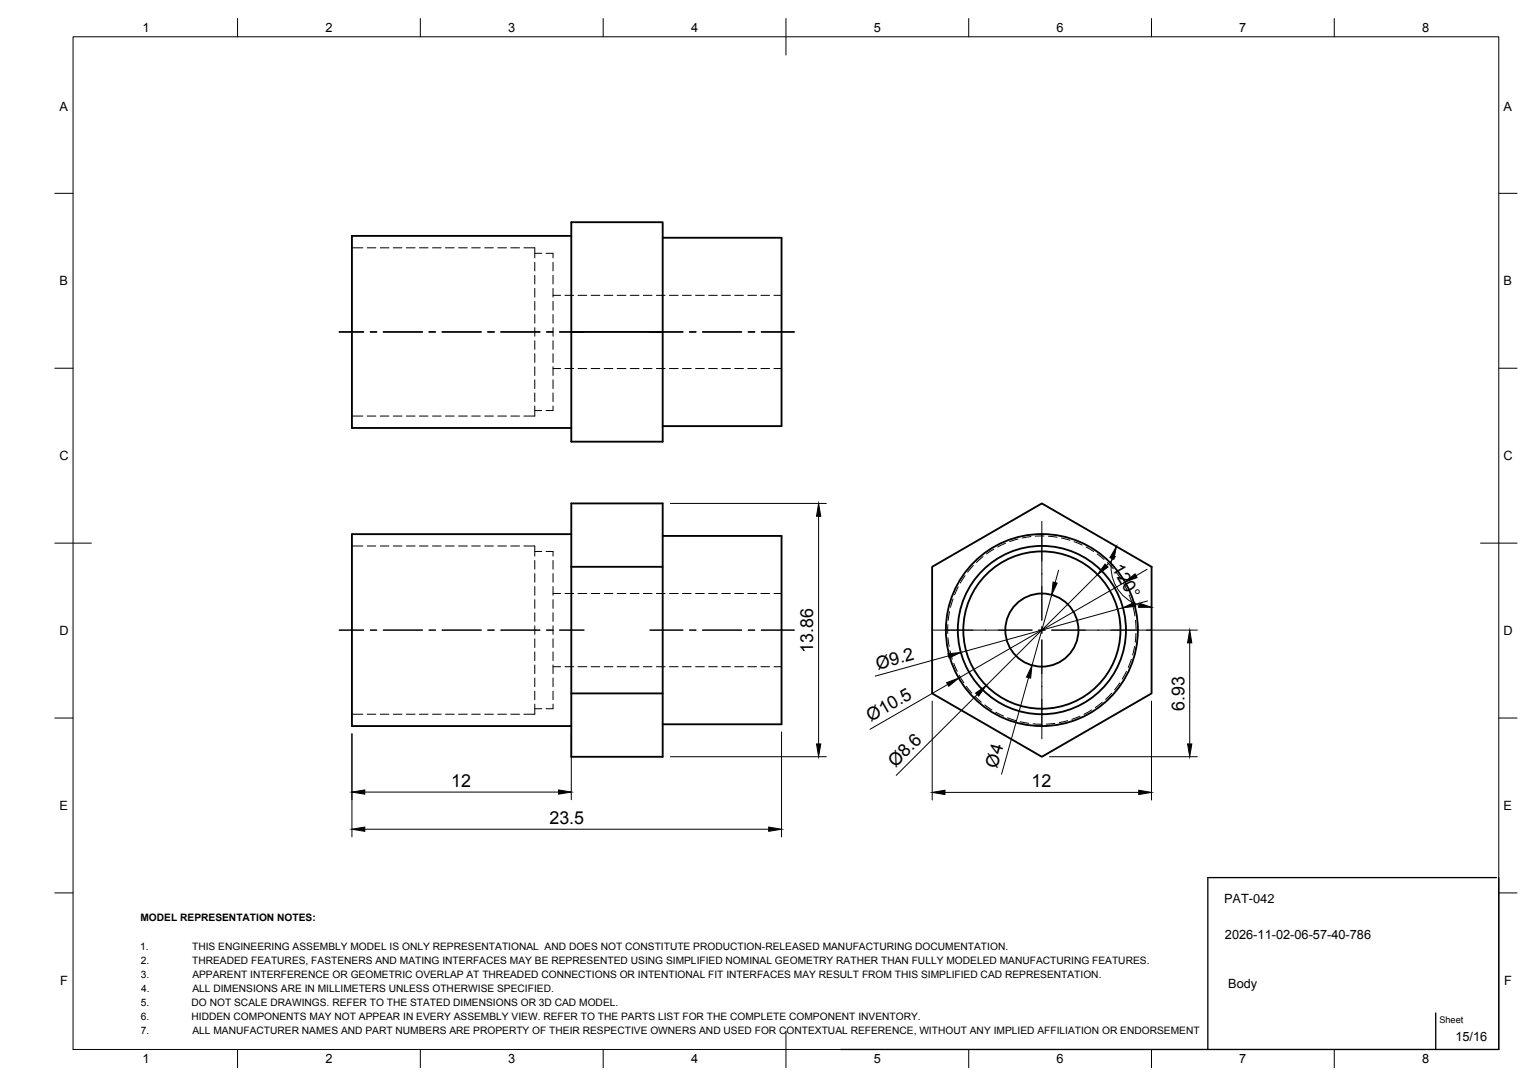
ISO-10303-21;
HEADER;
/* Generated by software containing ST-Developer
 * from STEP Tools, Inc. (www.steptools.com) 
 */

FILE_DESCRIPTION(
/* description */ ('Manifold and mounting hardware'),
/* implementation_level */ '2;1');

FILE_NAME(
/* name */ 'Body.step',
/* time_stamp */ '2026-10-28T21:46:49-07:00',
/* author */ (''),
/* organization */ (''),
/* preprocessor_version */ 'ST-DEVELOPER v20.2',
/* originating_system */ 'Autodesk Translation Framework v15.17.0.0',
/* authorisation */ '');

FILE_SCHEMA (('AUTOMOTIVE_DESIGN { 1 0 10303 214 3 1 1 }'));
ENDSEC;

DATA;
#10=MECHANICAL_DESIGN_GEOMETRIC_PRESENTATION_REPRESENTATION('',(#159),#5638);
#131=SHAPE_REPRESENTATION_RELATIONSHIP('SRR','None',#5711,#145);
#145=ADVANCED_BREP_SHAPE_REPRESENTATION('',(#173),#5633);
#159=STYLED_ITEM('',(#5839),#173);
#173=MANIFOLD_SOLID_BREP('Body1',#3149);
#241=FACE_BOUND('',#724,.T.);
#242=FACE_BOUND('',#726,.T.);
#243=FACE_BOUND('',#728,.T.);
#244=FACE_BOUND('',#736,.T.);
#245=FACE_BOUND('',#739,.T.);
#246=FACE_BOUND('',#743,.T.);
#318=CYLINDRICAL_SURFACE('',#3573,0.43);
#319=CYLINDRICAL_SURFACE('',#3590,0.46);
#320=CYLINDRICAL_SURFACE('',#3594,0.525);
#321=CYLINDRICAL_SURFACE('',#3595,0.515);
#322=CYLINDRICAL_SURFACE('',#3599,0.2);
#473=FACE_OUTER_BOUND('',#722,.T.);
#474=FACE_OUTER_BOUND('',#723,.T.);
#475=FACE_OUTER_BOUND('',#725,.T.);
#476=FACE_OUTER_BOUND('',#727,.T.);
#477=FACE_OUTER_BOUND('',#729,.T.);
#478=FACE_OUTER_BOUND('',#730,.T.);
#479=FACE_OUTER_BOUND('',#731,.T.);
#480=FACE_OUTER_BOUND('',#732,.T.);
#481=FACE_OUTER_BOUND('',#733,.T.);
#482=FACE_OUTER_BOUND('',#734,.T.);
#483=FACE_OUTER_BOUND('',#735,.T.);
#484=FACE_OUTER_BOUND('',#737,.T.);
#485=FACE_OUTER_BOUND('',#738,.T.);
#486=FACE_OUTER_BOUND('',#740,.T.);
#487=FACE_OUTER_BOUND('',#741,.T.);
#488=FACE_OUTER_BOUND('',#742,.T.);
#489=FACE_OUTER_BOUND('',#744,.T.);
#722=EDGE_LOOP('',(#2674,#2675,#2676,#2677));
#723=EDGE_LOOP('',(#2678));
#724=EDGE_LOOP('',(#2679));
#725=EDGE_LOOP('',(#2680,#2681,#2682,#2683,#2684,#2685));
#726=EDGE_LOOP('',(#2686));
#727=EDGE_LOOP('',(#2687,#2688,#2689,#2690,#2691,#2692));
#728=EDGE_LOOP('',(#2693));
#729=EDGE_LOOP('',(#2694,#2695,#2696,#2697));
#730=EDGE_LOOP('',(#2698,#2699,#2700,#2701));
#731=EDGE_LOOP('',(#2702,#2703,#2704,#2705));
#732=EDGE_LOOP('',(#2706,#2707,#2708,#2709));
#733=EDGE_LOOP('',(#2710,#2711,#2712,#2713));
#734=EDGE_LOOP('',(#2714,#2715,#2716,#2717));
#735=EDGE_LOOP('',(#2718));
#736=EDGE_LOOP('',(#2719));
#737=EDGE_LOOP('',(#2720,#2721,#2722,#2723));
#738=EDGE_LOOP('',(#2724));
#739=EDGE_LOOP('',(#2725));
#740=EDGE_LOOP('',(#2726,#2727,#2728,#2729));
#741=EDGE_LOOP('',(#2730,#2731,#2732,#2733));
#742=EDGE_LOOP('',(#2734));
#743=EDGE_LOOP('',(#2735));
#744=EDGE_LOOP('',(#2736,#2737,#2738,#2739));
#870=CIRCLE('',#3574,0.43);
#871=CIRCLE('',#3575,0.43);
#872=CIRCLE('',#3577,0.2);
#873=CIRCLE('',#3579,0.525);
#874=CIRCLE('',#3581,0.515);
#875=CIRCLE('',#3589,0.46);
#876=CIRCLE('',#3591,0.46);
#877=CIRCLE('',#3593,0.525);
#878=CIRCLE('',#3596,0.515);
#879=CIRCLE('',#3598,0.2);
#1099=LINE('',#5396,#1346);
#1100=LINE('',#5404,#1347);
#1101=LINE('',#5406,#1348);
#1102=LINE('',#5408,#1349);
#1103=LINE('',#5410,#1350);
#1104=LINE('',#5412,#1351);
#1105=LINE('',#5413,#1352);
#1106=LINE('',#5419,#1353);
#1107=LINE('',#5421,#1354);
#1108=LINE('',#5423,#1355);
#1109=LINE('',#5425,#1356);
#1110=LINE('',#5427,#1357);
#1111=LINE('',#5428,#1358);
#1112=LINE('',#5432,#1359);
#1113=LINE('',#5433,#1360);
#1114=LINE('',#5435,#1361);
#1115=LINE('',#5437,#1362);
#1116=LINE('',#5439,#1363);
#1117=LINE('',#5441,#1364);
#1118=LINE('',#5448,#1365);
#1119=LINE('',#5454,#1366);
#1120=LINE('',#5458,#1367);
#1121=LINE('',#5463,#1368);
#1346=VECTOR('',#4406,0.43);
#1347=VECTOR('',#4415,1.);
#1348=VECTOR('',#4416,1.);
#1349=VECTOR('',#4417,1.);
#1350=VECTOR('',#4418,1.);
#1351=VECTOR('',#4419,1.);
#1352=VECTOR('',#4420,1.);
#1353=VECTOR('',#4425,1.);
#1354=VECTOR('',#4426,1.);
#1355=VECTOR('',#4427,1.);
#1356=VECTOR('',#4428,1.);
#1357=VECTOR('',#4429,1.);
#1358=VECTOR('',#4430,1.);
#1359=VECTOR('',#4435,1.);
#1360=VECTOR('',#4436,1.);
#1361=VECTOR('',#4439,1.);
#1362=VECTOR('',#4442,1.);
#1363=VECTOR('',#4445,1.);
#1364=VECTOR('',#4448,1.);
#1365=VECTOR('',#4457,0.46);
#1366=VECTOR('',#4466,0.525);
#1367=VECTOR('',#4471,0.515);
#1368=VECTOR('',#4478,0.2);
#1600=VERTEX_POINT('',#5393);
#1601=VERTEX_POINT('',#5395);
#1602=VERTEX_POINT('',#5399);
#1603=VERTEX_POINT('',#5402);
#1604=VERTEX_POINT('',#5403);
#1605=VERTEX_POINT('',#5405);
#1606=VERTEX_POINT('',#5407);
#1607=VERTEX_POINT('',#5409);
#1608=VERTEX_POINT('',#5411);
#1609=VERTEX_POINT('',#5414);
#1610=VERTEX_POINT('',#5417);
#1611=VERTEX_POINT('',#5418);
#1612=VERTEX_POINT('',#5420);
#1613=VERTEX_POINT('',#5422);
#1614=VERTEX_POINT('',#5424);
#1615=VERTEX_POINT('',#5426);
#1616=VERTEX_POINT('',#5429);
#1617=VERTEX_POINT('',#5444);
#1618=VERTEX_POINT('',#5447);
#1619=VERTEX_POINT('',#5451);
#1620=VERTEX_POINT('',#5456);
#1621=VERTEX_POINT('',#5460);
#1966=EDGE_CURVE('',#1600,#1600,#870,.T.);
#1967=EDGE_CURVE('',#1600,#1601,#1099,.T.);
#1968=EDGE_CURVE('',#1601,#1601,#871,.T.);
#1969=EDGE_CURVE('',#1602,#1602,#872,.T.);
#1970=EDGE_CURVE('',#1603,#1604,#1100,.T.);
#1971=EDGE_CURVE('',#1604,#1605,#1101,.T.);
#1972=EDGE_CURVE('',#1605,#1606,#1102,.T.);
#1973=EDGE_CURVE('',#1606,#1607,#1103,.T.);
#1974=EDGE_CURVE('',#1607,#1608,#1104,.T.);
#1975=EDGE_CURVE('',#1608,#1603,#1105,.T.);
#1976=EDGE_CURVE('',#1609,#1609,#873,.T.);
#1977=EDGE_CURVE('',#1610,#1611,#1106,.T.);
#1978=EDGE_CURVE('',#1612,#1610,#1107,.T.);
#1979=EDGE_CURVE('',#1613,#1612,#1108,.T.);
#1980=EDGE_CURVE('',#1614,#1613,#1109,.T.);
#1981=EDGE_CURVE('',#1615,#1614,#1110,.T.);
#1982=EDGE_CURVE('',#1611,#1615,#1111,.T.);
#1983=EDGE_CURVE('',#1616,#1616,#874,.T.);
#1984=EDGE_CURVE('',#1610,#1603,#1112,.T.);
#1985=EDGE_CURVE('',#1612,#1608,#1113,.T.);
#1986=EDGE_CURVE('',#1613,#1607,#1114,.T.);
#1987=EDGE_CURVE('',#1614,#1606,#1115,.T.);
#1988=EDGE_CURVE('',#1615,#1605,#1116,.T.);
#1989=EDGE_CURVE('',#1611,#1604,#1117,.T.);
#1990=EDGE_CURVE('',#1617,#1617,#875,.T.);
#1991=EDGE_CURVE('',#1617,#1618,#1118,.T.);
#1992=EDGE_CURVE('',#1618,#1618,#876,.T.);
#1993=EDGE_CURVE('',#1619,#1619,#877,.T.);
#1994=EDGE_CURVE('',#1609,#1619,#1119,.T.);
#1995=EDGE_CURVE('',#1620,#1620,#878,.T.);
#1996=EDGE_CURVE('',#1620,#1616,#1120,.T.);
#1997=EDGE_CURVE('',#1621,#1621,#879,.T.);
#1998=EDGE_CURVE('',#1621,#1602,#1121,.T.);
#2674=ORIENTED_EDGE('',*,*,#1966,.F.);
#2675=ORIENTED_EDGE('',*,*,#1967,.T.);
#2676=ORIENTED_EDGE('',*,*,#1968,.F.);
#2677=ORIENTED_EDGE('',*,*,#1967,.F.);
#2678=ORIENTED_EDGE('',*,*,#1966,.T.);
#2679=ORIENTED_EDGE('',*,*,#1969,.F.);
#2680=ORIENTED_EDGE('',*,*,#1970,.T.);
#2681=ORIENTED_EDGE('',*,*,#1971,.T.);
#2682=ORIENTED_EDGE('',*,*,#1972,.T.);
#2683=ORIENTED_EDGE('',*,*,#1973,.T.);
#2684=ORIENTED_EDGE('',*,*,#1974,.T.);
#2685=ORIENTED_EDGE('',*,*,#1975,.T.);
#2686=ORIENTED_EDGE('',*,*,#1976,.T.);
#2687=ORIENTED_EDGE('',*,*,#1977,.F.);
#2688=ORIENTED_EDGE('',*,*,#1978,.F.);
#2689=ORIENTED_EDGE('',*,*,#1979,.F.);
#2690=ORIENTED_EDGE('',*,*,#1980,.F.);
#2691=ORIENTED_EDGE('',*,*,#1981,.F.);
#2692=ORIENTED_EDGE('',*,*,#1982,.F.);
#2693=ORIENTED_EDGE('',*,*,#1983,.F.);
#2694=ORIENTED_EDGE('',*,*,#1978,.T.);
#2695=ORIENTED_EDGE('',*,*,#1984,.T.);
#2696=ORIENTED_EDGE('',*,*,#1975,.F.);
#2697=ORIENTED_EDGE('',*,*,#1985,.F.);
#2698=ORIENTED_EDGE('',*,*,#1979,.T.);
#2699=ORIENTED_EDGE('',*,*,#1985,.T.);
#2700=ORIENTED_EDGE('',*,*,#1974,.F.);
#2701=ORIENTED_EDGE('',*,*,#1986,.F.);
#2702=ORIENTED_EDGE('',*,*,#1980,.T.);
#2703=ORIENTED_EDGE('',*,*,#1986,.T.);
#2704=ORIENTED_EDGE('',*,*,#1973,.F.);
#2705=ORIENTED_EDGE('',*,*,#1987,.F.);
#2706=ORIENTED_EDGE('',*,*,#1981,.T.);
#2707=ORIENTED_EDGE('',*,*,#1987,.T.);
#2708=ORIENTED_EDGE('',*,*,#1972,.F.);
#2709=ORIENTED_EDGE('',*,*,#1988,.F.);
#2710=ORIENTED_EDGE('',*,*,#1982,.T.);
#2711=ORIENTED_EDGE('',*,*,#1988,.T.);
#2712=ORIENTED_EDGE('',*,*,#1971,.F.);
#2713=ORIENTED_EDGE('',*,*,#1989,.F.);
#2714=ORIENTED_EDGE('',*,*,#1977,.T.);
#2715=ORIENTED_EDGE('',*,*,#1989,.T.);
#2716=ORIENTED_EDGE('',*,*,#1970,.F.);
#2717=ORIENTED_EDGE('',*,*,#1984,.F.);
#2718=ORIENTED_EDGE('',*,*,#1990,.F.);
#2719=ORIENTED_EDGE('',*,*,#1968,.T.);
#2720=ORIENTED_EDGE('',*,*,#1990,.T.);
#2721=ORIENTED_EDGE('',*,*,#1991,.T.);
#2722=ORIENTED_EDGE('',*,*,#1992,.F.);
#2723=ORIENTED_EDGE('',*,*,#1991,.F.);
#2724=ORIENTED_EDGE('',*,*,#1993,.F.);
#2725=ORIENTED_EDGE('',*,*,#1992,.T.);
#2726=ORIENTED_EDGE('',*,*,#1976,.F.);
#2727=ORIENTED_EDGE('',*,*,#1994,.T.);
#2728=ORIENTED_EDGE('',*,*,#1993,.T.);
#2729=ORIENTED_EDGE('',*,*,#1994,.F.);
#2730=ORIENTED_EDGE('',*,*,#1995,.F.);
#2731=ORIENTED_EDGE('',*,*,#1996,.T.);
#2732=ORIENTED_EDGE('',*,*,#1983,.T.);
#2733=ORIENTED_EDGE('',*,*,#1996,.F.);
#2734=ORIENTED_EDGE('',*,*,#1995,.T.);
#2735=ORIENTED_EDGE('',*,*,#1997,.F.);
#2736=ORIENTED_EDGE('',*,*,#1997,.T.);
#2737=ORIENTED_EDGE('',*,*,#1998,.T.);
#2738=ORIENTED_EDGE('',*,*,#1969,.T.);
#2739=ORIENTED_EDGE('',*,*,#1998,.F.);
#2927=PLANE('',#3576);
#2928=PLANE('',#3578);
#2929=PLANE('',#3580);
#2930=PLANE('',#3582);
#2931=PLANE('',#3583);
#2932=PLANE('',#3584);
#2933=PLANE('',#3585);
#2934=PLANE('',#3586);
#2935=PLANE('',#3587);
#2936=PLANE('',#3588);
#2937=PLANE('',#3592);
#2938=PLANE('',#3597);
#3097=ADVANCED_FACE('',(#473),#318,.F.);
#3098=ADVANCED_FACE('',(#474,#241),#2927,.T.);
#3099=ADVANCED_FACE('',(#475,#242),#2928,.T.);
#3100=ADVANCED_FACE('',(#476,#243),#2929,.F.);
#3101=ADVANCED_FACE('',(#477),#2930,.T.);
#3102=ADVANCED_FACE('',(#478),#2931,.T.);
#3103=ADVANCED_FACE('',(#479),#2932,.T.);
#3104=ADVANCED_FACE('',(#480),#2933,.T.);
#3105=ADVANCED_FACE('',(#481),#2934,.T.);
#3106=ADVANCED_FACE('',(#482),#2935,.T.);
#3107=ADVANCED_FACE('',(#483,#244),#2936,.T.);
#3108=ADVANCED_FACE('',(#484),#319,.F.);
#3109=ADVANCED_FACE('',(#485,#245),#2937,.T.);
#3110=ADVANCED_FACE('',(#486),#320,.T.);
#3111=ADVANCED_FACE('',(#487),#321,.T.);
#3112=ADVANCED_FACE('',(#488,#246),#2938,.T.);
#3113=ADVANCED_FACE('',(#489),#322,.F.);
#3149=CLOSED_SHELL('',(#3097,#3098,#3099,#3100,#3101,#3102,#3103,#3104,
#3105,#3106,#3107,#3108,#3109,#3110,#3111,#3112,#3113));
#3572=AXIS2_PLACEMENT_3D('',#5391,#4400,#4401);
#3573=AXIS2_PLACEMENT_3D('',#5392,#4402,#4403);
#3574=AXIS2_PLACEMENT_3D('',#5394,#4404,#4405);
#3575=AXIS2_PLACEMENT_3D('',#5397,#4407,#4408);
#3576=AXIS2_PLACEMENT_3D('',#5398,#4409,#4410);
#3577=AXIS2_PLACEMENT_3D('',#5400,#4411,#4412);
#3578=AXIS2_PLACEMENT_3D('',#5401,#4413,#4414);
#3579=AXIS2_PLACEMENT_3D('',#5415,#4421,#4422);
#3580=AXIS2_PLACEMENT_3D('',#5416,#4423,#4424);
#3581=AXIS2_PLACEMENT_3D('',#5430,#4431,#4432);
#3582=AXIS2_PLACEMENT_3D('',#5431,#4433,#4434);
#3583=AXIS2_PLACEMENT_3D('',#5434,#4437,#4438);
#3584=AXIS2_PLACEMENT_3D('',#5436,#4440,#4441);
#3585=AXIS2_PLACEMENT_3D('',#5438,#4443,#4444);
#3586=AXIS2_PLACEMENT_3D('',#5440,#4446,#4447);
#3587=AXIS2_PLACEMENT_3D('',#5442,#4449,#4450);
#3588=AXIS2_PLACEMENT_3D('',#5443,#4451,#4452);
#3589=AXIS2_PLACEMENT_3D('',#5445,#4453,#4454);
#3590=AXIS2_PLACEMENT_3D('',#5446,#4455,#4456);
#3591=AXIS2_PLACEMENT_3D('',#5449,#4458,#4459);
#3592=AXIS2_PLACEMENT_3D('',#5450,#4460,#4461);
#3593=AXIS2_PLACEMENT_3D('',#5452,#4462,#4463);
#3594=AXIS2_PLACEMENT_3D('',#5453,#4464,#4465);
#3595=AXIS2_PLACEMENT_3D('',#5455,#4467,#4468);
#3596=AXIS2_PLACEMENT_3D('',#5457,#4469,#4470);
#3597=AXIS2_PLACEMENT_3D('',#5459,#4472,#4473);
#3598=AXIS2_PLACEMENT_3D('',#5461,#4474,#4475);
#3599=AXIS2_PLACEMENT_3D('',#5462,#4476,#4477);
#4400=DIRECTION('axis',(0.,0.,1.));
#4401=DIRECTION('refdir',(1.,0.,0.));
#4402=DIRECTION('center_axis',(0.,1.,0.));
#4403=DIRECTION('ref_axis',(1.,0.,0.));
#4404=DIRECTION('center_axis',(0.,1.,0.));
#4405=DIRECTION('ref_axis',(1.,0.,0.));
#4406=DIRECTION('',(0.,1.,0.));
#4407=DIRECTION('center_axis',(0.,-1.,0.));
#4408=DIRECTION('ref_axis',(1.,0.,0.));
#4409=DIRECTION('center_axis',(0.,1.,0.));
#4410=DIRECTION('ref_axis',(1.,0.,0.));
#4411=DIRECTION('center_axis',(0.,1.,0.));
#4412=DIRECTION('ref_axis',(1.,0.,0.));
#4413=DIRECTION('center_axis',(0.,1.,0.));
#4414=DIRECTION('ref_axis',(1.,0.,0.));
#4415=DIRECTION('',(0.5,0.,-0.866025403784439));
#4416=DIRECTION('',(-0.5,0.,-0.866025403784439));
#4417=DIRECTION('',(-1.,0.,-1.60246890531964E-16));
#4418=DIRECTION('',(-0.5,0.,0.866025403784439));
#4419=DIRECTION('',(0.5,0.,0.866025403784439));
#4420=DIRECTION('',(1.,0.,1.60246890531964E-16));
#4421=DIRECTION('center_axis',(0.,-1.,0.));
#4422=DIRECTION('ref_axis',(1.,0.,0.));
#4423=DIRECTION('center_axis',(0.,1.,0.));
#4424=DIRECTION('ref_axis',(1.,0.,0.));
#4425=DIRECTION('',(0.5,0.,-0.866025403784439));
#4426=DIRECTION('',(1.,0.,1.60246890531964E-16));
#4427=DIRECTION('',(0.5,0.,0.866025403784439));
#4428=DIRECTION('',(-0.5,0.,0.866025403784439));
#4429=DIRECTION('',(-1.,0.,-1.60246890531964E-16));
#4430=DIRECTION('',(-0.5,0.,-0.866025403784439));
#4431=DIRECTION('center_axis',(0.,-1.,0.));
#4432=DIRECTION('ref_axis',(1.,0.,0.));
#4433=DIRECTION('center_axis',(-1.60246890531964E-16,0.,1.));
#4434=DIRECTION('ref_axis',(1.,0.,1.60246890531964E-16));
#4435=DIRECTION('',(0.,1.,0.));
#4436=DIRECTION('',(0.,1.,0.));
#4437=DIRECTION('center_axis',(-0.866025403784439,0.,0.5));
#4438=DIRECTION('ref_axis',(0.5,0.,0.866025403784439));
#4439=DIRECTION('',(0.,1.,0.));
#4440=DIRECTION('center_axis',(-0.866025403784439,0.,-0.5));
#4441=DIRECTION('ref_axis',(-0.5,0.,0.866025403784439));
#4442=DIRECTION('',(0.,1.,0.));
#4443=DIRECTION('center_axis',(1.60246890531964E-16,0.,-1.));
#4444=DIRECTION('ref_axis',(-1.,0.,-1.60246890531964E-16));
#4445=DIRECTION('',(0.,1.,0.));
#4446=DIRECTION('center_axis',(0.866025403784439,0.,-0.5));
#4447=DIRECTION('ref_axis',(-0.5,0.,-0.866025403784439));
#4448=DIRECTION('',(0.,1.,0.));
#4449=DIRECTION('center_axis',(0.866025403784439,0.,0.5));
#4450=DIRECTION('ref_axis',(0.5,0.,-0.866025403784439));
#4451=DIRECTION('center_axis',(0.,1.,0.));
#4452=DIRECTION('ref_axis',(0.,0.,1.));
#4453=DIRECTION('center_axis',(0.,-1.,0.));
#4454=DIRECTION('ref_axis',(1.,0.,0.));
#4455=DIRECTION('center_axis',(0.,-1.,0.));
#4456=DIRECTION('ref_axis',(1.,0.,0.));
#4457=DIRECTION('',(0.,1.,0.));
#4458=DIRECTION('center_axis',(0.,-1.,0.));
#4459=DIRECTION('ref_axis',(1.,0.,0.));
#4460=DIRECTION('center_axis',(0.,1.,0.));
#4461=DIRECTION('ref_axis',(0.,0.,1.));
#4462=DIRECTION('center_axis',(0.,-1.,0.));
#4463=DIRECTION('ref_axis',(1.,0.,0.));
#4464=DIRECTION('center_axis',(0.,-1.,0.));
#4465=DIRECTION('ref_axis',(1.,0.,0.));
#4466=DIRECTION('',(0.,1.,0.));
#4467=DIRECTION('center_axis',(0.,-1.,0.));
#4468=DIRECTION('ref_axis',(1.,0.,0.));
#4469=DIRECTION('center_axis',(0.,-1.,0.));
#4470=DIRECTION('ref_axis',(1.,0.,0.));
#4471=DIRECTION('',(0.,1.,0.));
#4472=DIRECTION('center_axis',(0.,-1.,0.));
#4473=DIRECTION('ref_axis',(0.,0.,-1.));
#4474=DIRECTION('center_axis',(0.,-1.,0.));
#4475=DIRECTION('ref_axis',(1.,0.,0.));
#4476=DIRECTION('center_axis',(0.,-1.,0.));
#4477=DIRECTION('ref_axis',(1.,0.,0.));
#4478=DIRECTION('',(0.,1.,0.));
#5391=CARTESIAN_POINT('',(0.,0.,0.));
#5392=CARTESIAN_POINT('Origin',(0.,0.6,0.));
#5393=CARTESIAN_POINT('',(-0.43,0.6,5.26598123633362E-17));
#5394=CARTESIAN_POINT('Origin',(0.,0.6,0.));
#5395=CARTESIAN_POINT('',(-0.43,0.7,-5.26598123633362E-17));
#5396=CARTESIAN_POINT('',(-0.43,0.6,5.26598123633362E-17));
#5397=CARTESIAN_POINT('Origin',(0.,0.7,0.));
#5398=CARTESIAN_POINT('Origin',(0.,0.6,0.));
#5399=CARTESIAN_POINT('',(-0.2,0.6,2.44929359829471E-17));
#5400=CARTESIAN_POINT('Origin',(0.,0.6,0.));
#5401=CARTESIAN_POINT('Origin',(0.,0.5,-1.11022302462516E-16));
#5402=CARTESIAN_POINT('',(0.346410161513776,0.5,0.6));
#5403=CARTESIAN_POINT('',(0.692820323027551,0.5,0.));
#5404=CARTESIAN_POINT('',(0.346410161513776,0.5,0.6));
#5405=CARTESIAN_POINT('',(0.346410161513776,0.5,-0.6));
#5406=CARTESIAN_POINT('',(0.692820323027551,0.5,0.));
#5407=CARTESIAN_POINT('',(-0.346410161513775,0.5,-0.6));
#5408=CARTESIAN_POINT('',(0.346410161513776,0.5,-0.6));
#5409=CARTESIAN_POINT('',(-0.692820323027551,0.5,-8.48460190979926E-17));
#5410=CARTESIAN_POINT('',(-0.346410161513775,0.5,-0.6));
#5411=CARTESIAN_POINT('',(-0.346410161513776,0.5,0.6));
#5412=CARTESIAN_POINT('',(-0.692820323027551,0.5,-8.48460190979926E-17));
#5413=CARTESIAN_POINT('',(-0.346410161513776,0.5,0.6));
#5414=CARTESIAN_POINT('',(-0.525,0.5,-6.4293956955236E-17));
#5415=CARTESIAN_POINT('Origin',(0.,0.5,0.));
#5416=CARTESIAN_POINT('Origin',(0.,0.,-1.11022302462516E-16));
#5417=CARTESIAN_POINT('',(0.346410161513776,0.,0.6));
#5418=CARTESIAN_POINT('',(0.692820323027551,0.,0.));
#5419=CARTESIAN_POINT('',(0.346410161513776,0.,0.6));
#5420=CARTESIAN_POINT('',(-0.346410161513776,0.,0.6));
#5421=CARTESIAN_POINT('',(-0.346410161513776,0.,0.6));
#5422=CARTESIAN_POINT('',(-0.692820323027551,0.,-8.48460190979926E-17));
#5423=CARTESIAN_POINT('',(-0.692820323027551,0.,-8.48460190979926E-17));
#5424=CARTESIAN_POINT('',(-0.346410161513775,0.,-0.6));
#5425=CARTESIAN_POINT('',(-0.346410161513775,0.,-0.6));
#5426=CARTESIAN_POINT('',(0.346410161513776,0.,-0.6));
#5427=CARTESIAN_POINT('',(0.346410161513776,0.,-0.6));
#5428=CARTESIAN_POINT('',(0.692820323027551,0.,0.));
#5429=CARTESIAN_POINT('',(-0.515,0.,-6.30693101560887E-17));
#5430=CARTESIAN_POINT('Origin',(0.,0.,0.));
#5431=CARTESIAN_POINT('Origin',(-0.346410161513776,0.,0.6));
#5432=CARTESIAN_POINT('',(0.346410161513776,0.,0.6));
#5433=CARTESIAN_POINT('',(-0.346410161513776,0.,0.6));
#5434=CARTESIAN_POINT('Origin',(-0.692820323027551,0.,-8.48460190979926E-17));
#5435=CARTESIAN_POINT('',(-0.692820323027551,0.,-8.48460190979926E-17));
#5436=CARTESIAN_POINT('Origin',(-0.346410161513775,0.,-0.6));
#5437=CARTESIAN_POINT('',(-0.346410161513775,0.,-0.6));
#5438=CARTESIAN_POINT('Origin',(0.346410161513776,0.,-0.6));
#5439=CARTESIAN_POINT('',(0.346410161513776,0.,-0.6));
#5440=CARTESIAN_POINT('Origin',(0.692820323027551,0.,0.));
#5441=CARTESIAN_POINT('',(0.692820323027551,0.,0.));
#5442=CARTESIAN_POINT('Origin',(0.346410161513776,0.,0.6));
#5443=CARTESIAN_POINT('Origin',(0.46,0.7,0.));
#5444=CARTESIAN_POINT('',(-0.46,0.7,-5.63337527607782E-17));
#5445=CARTESIAN_POINT('Origin',(0.,0.7,0.));
#5446=CARTESIAN_POINT('Origin',(0.,1.2,0.));
#5447=CARTESIAN_POINT('',(-0.46,1.7,-5.63337527607782E-17));
#5448=CARTESIAN_POINT('',(-0.46,1.2,-5.63337527607782E-17));
#5449=CARTESIAN_POINT('Origin',(0.,1.7,0.));
#5450=CARTESIAN_POINT('Origin',(0.525,1.7,0.));
#5451=CARTESIAN_POINT('',(-0.525,1.7,-6.4293956955236E-17));
#5452=CARTESIAN_POINT('Origin',(0.,1.7,0.));
#5453=CARTESIAN_POINT('Origin',(0.,1.1,0.));
#5454=CARTESIAN_POINT('',(-0.525,1.1,-6.4293956955236E-17));
#5455=CARTESIAN_POINT('Origin',(0.,-0.325,0.));
#5456=CARTESIAN_POINT('',(-0.515,-0.65,-6.30693101560887E-17));
#5457=CARTESIAN_POINT('Origin',(0.,-0.65,0.));
#5458=CARTESIAN_POINT('',(-0.515,-0.325,-6.30693101560887E-17));
#5459=CARTESIAN_POINT('Origin',(0.2,-0.65,0.));
#5460=CARTESIAN_POINT('',(-0.2,-0.65,-2.44929359829471E-17));
#5461=CARTESIAN_POINT('Origin',(0.,-0.65,0.));
#5462=CARTESIAN_POINT('Origin',(0.,0.0249999999999999,0.));
#5463=CARTESIAN_POINT('',(-0.2,0.0249999999999999,-2.44929359829471E-17));
#5616=UNCERTAINTY_MEASURE_WITH_UNIT(LENGTH_MEASURE(0.001),#5639,
'DISTANCE_ACCURACY_VALUE',
'Maximum model space distance between geometric entities at asserted c
onnectivities');
#5621=UNCERTAINTY_MEASURE_WITH_UNIT(LENGTH_MEASURE(0.001),#5639,
'DISTANCE_ACCURACY_VALUE',
'Maximum model space distance between geometric entities at asserted c
onnectivities');
#5633=(
GEOMETRIC_REPRESENTATION_CONTEXT(3)
GLOBAL_UNCERTAINTY_ASSIGNED_CONTEXT((#5616))
GLOBAL_UNIT_ASSIGNED_CONTEXT((#5639,#5641,#5642))
REPRESENTATION_CONTEXT('','3D')
);
#5638=(
GEOMETRIC_REPRESENTATION_CONTEXT(3)
GLOBAL_UNCERTAINTY_ASSIGNED_CONTEXT((#5621))
GLOBAL_UNIT_ASSIGNED_CONTEXT((#5639,#5641,#5642))
REPRESENTATION_CONTEXT('','3D')
);
#5639=(
LENGTH_UNIT()
NAMED_UNIT(*)
SI_UNIT(.CENTI.,.METRE.)
);
#5641=(
NAMED_UNIT(*)
PLANE_ANGLE_UNIT()
SI_UNIT($,.RADIAN.)
);
#5642=(
NAMED_UNIT(*)
SI_UNIT($,.STERADIAN.)
SOLID_ANGLE_UNIT()
);
#5654=SHAPE_DEFINITION_REPRESENTATION(#5670,#5711);
#5670=PRODUCT_DEFINITION_SHAPE('',$,#5728);
#5711=SHAPE_REPRESENTATION('',(#3572),#5633);
#5716=PRODUCT_DEFINITION_CONTEXT('part definition',#5766,'design');
#5728=PRODUCT_DEFINITION('Body','Body',#5744,#5716);
#5744=PRODUCT_DEFINITION_FORMATION('',$,#5779);
#5766=APPLICATION_CONTEXT(
'Core Data for Automotive Mechanical Design Process');
#5767=PRODUCT_CONTEXT('part definition',#5766,'mechanical');
#5779=PRODUCT('Body','Body','Body',(#5767));
#5833=COLOUR_RGB('Dark Blue',0.08,0.2,0.34);
#5834=FILL_AREA_STYLE_COLOUR('',#5833);
#5835=FILL_AREA_STYLE('',(#5834));
#5836=SURFACE_STYLE_FILL_AREA(#5835);
#5837=SURFACE_SIDE_STYLE('',(#5836));
#5838=SURFACE_STYLE_USAGE(.BOTH.,#5837);
#5839=PRESENTATION_STYLE_ASSIGNMENT((#5838));
ENDSEC;
END-ISO-10303-21;
